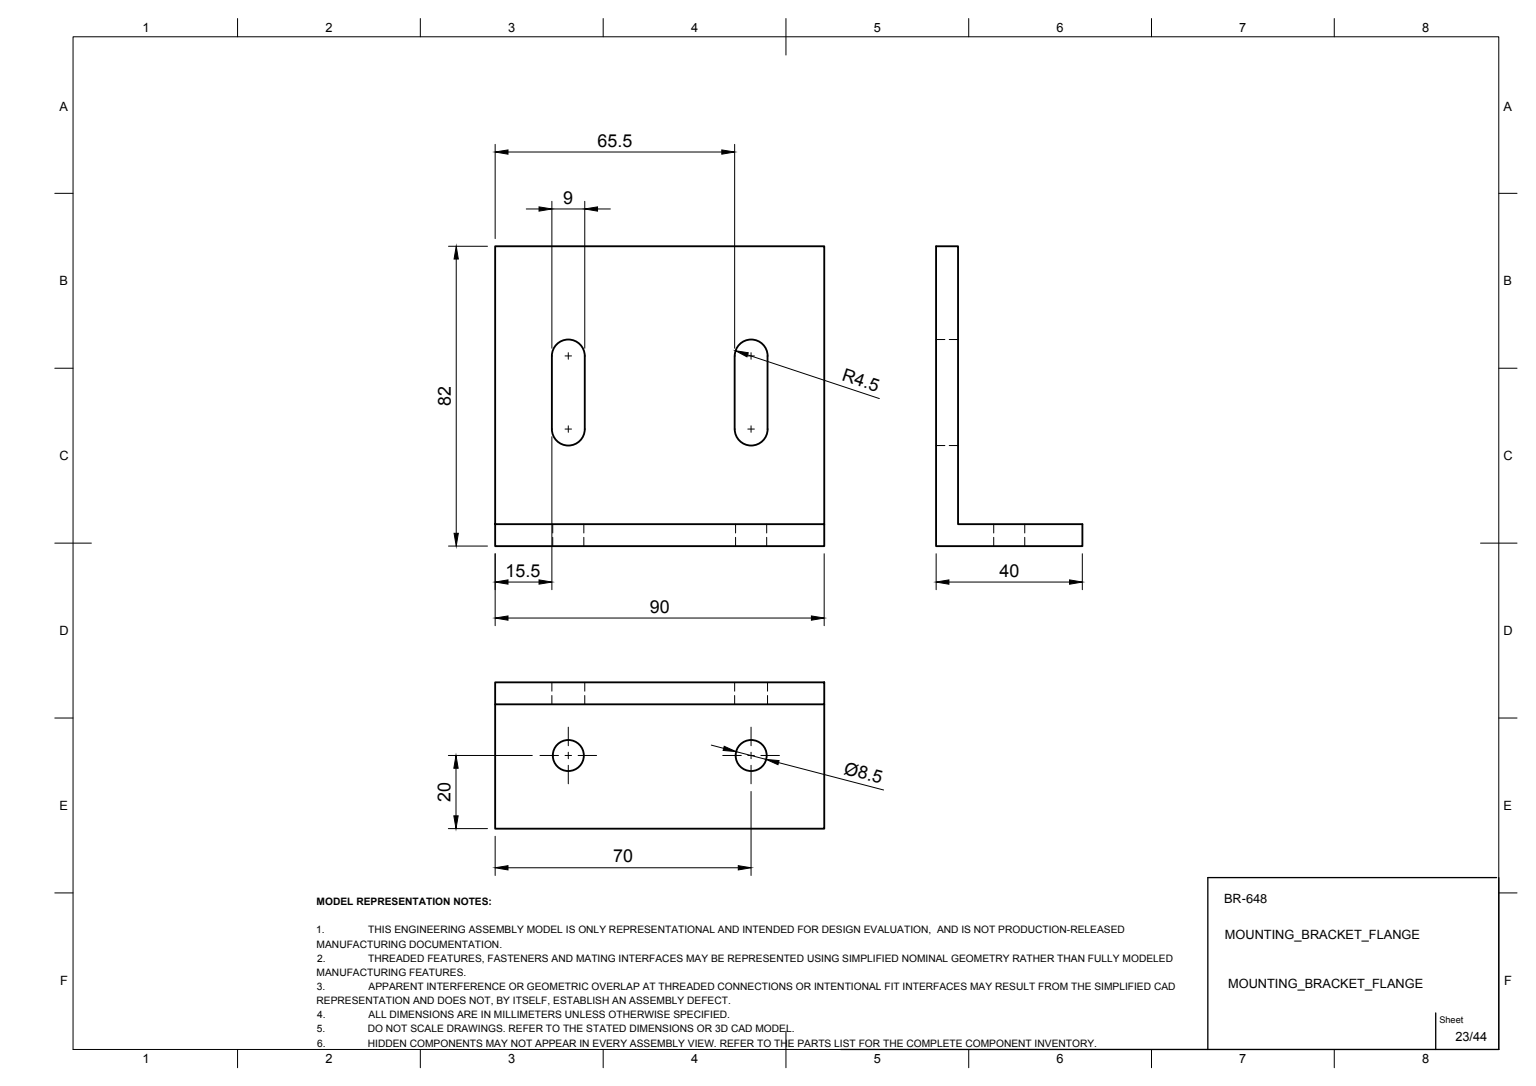
ISO-10303-21;
HEADER;
FILE_DESCRIPTION((''),'2;1');
FILE_NAME('MOUNTING_BRACKET_FLANGE.step','2026-10-01T22:05:39-07:00',(''),(''),'','','');
FILE_SCHEMA (('AUTOMOTIVE_DESIGN { 1 0 10303 214 3 1 1 }'));
ENDSEC;
DATA;
#10=MECHANICAL_DESIGN_GEOMETRIC_PRESENTATION_REPRESENTATION('',(#623),#24628);
#539=SHAPE_REPRESENTATION_RELATIONSHIP('SRR','None',#24811,#581) ;
#581=ADVANCED_BREP_SHAPE_REPRESENTATION('',(#662),#24601) ;
#623=STYLED_ITEM('',(#25037),#662) ;
#662=MANIFOLD_SOLID_BREP('MOUNTING_BRACKET_FLANGE',#13165) ;
#863=FACE_BOUND('',#4382,.T.) ;
#864=FACE_BOUND('',#4383,.T.) ;
#865=FACE_BOUND('',#4386,.T.) ;
#866=FACE_BOUND('',#4387,.T.) ;
#867=FACE_BOUND('',#4390,.T.) ;
#868=FACE_BOUND('',#4391,.T.) ;
#869=FACE_BOUND('',#4394,.T.) ;
#870=FACE_BOUND('',#4395,.T.) ;
#1406=LINE('',#22245,#2242) ;
#1407=LINE('',#22248,#2243) ;
#1408=LINE('',#22251,#2244) ;
#1409=LINE('',#22253,#2245) ;
#1410=LINE('',#22254,#2246) ;
#1411=LINE('',#22260,#2247) ;
#1412=LINE('',#22262,#2248) ;
#1413=LINE('',#22263,#2249) ;
#1414=LINE('',#22268,#2250) ;
#1415=LINE('',#22275,#2251) ;
#1416=LINE('',#22278,#2252) ;
#1417=LINE('',#22281,#2253) ;
#1418=LINE('',#22283,#2254) ;
#1419=LINE('',#22284,#2255) ;
#1420=LINE('',#22290,#2256) ;
#1421=LINE('',#22292,#2257) ;
#1422=LINE('',#22293,#2258) ;
#1423=LINE('',#22298,#2259) ;
#1424=LINE('',#22303,#2260) ;
#1425=LINE('',#22305,#2261) ;
#1426=LINE('',#22307,#2262) ;
#1427=LINE('',#22308,#2263) ;
#1428=LINE('',#22311,#2264) ;
#1429=LINE('',#22313,#2265) ;
#1430=LINE('',#22314,#2266) ;
#1431=LINE('',#22317,#2267) ;
#1432=LINE('',#22319,#2268) ;
#1433=LINE('',#22320,#2269) ;
#1434=LINE('',#22324,#2270) ;
#1435=LINE('',#22325,#2271) ;
#1436=LINE('',#22326,#2272) ;
#1437=LINE('',#22329,#2273) ;
#1438=LINE('',#22330,#2274) ;
#1439=LINE('',#22333,#2275) ;
#1440=LINE('',#22334,#2276) ;
#1441=LINE('',#22336,#2277) ;
#2242=VECTOR('',#18101,1.) ;
#2243=VECTOR('',#18104,1.) ;
#2244=VECTOR('',#18107,1.) ;
#2245=VECTOR('',#18108,1.) ;
#2246=VECTOR('',#18109,1.) ;
#2247=VECTOR('',#18116,1.) ;
#2248=VECTOR('',#18119,1.) ;
#2249=VECTOR('',#18120,1.) ;
#2250=VECTOR('',#18125,0.425) ;
#2251=VECTOR('',#18132,1.) ;
#2252=VECTOR('',#18135,1.) ;
#2253=VECTOR('',#18138,1.) ;
#2254=VECTOR('',#18139,1.) ;
#2255=VECTOR('',#18140,1.) ;
#2256=VECTOR('',#18147,1.) ;
#2257=VECTOR('',#18150,1.) ;
#2258=VECTOR('',#18151,1.) ;
#2259=VECTOR('',#18156,0.425) ;
#2260=VECTOR('',#18161,1.) ;
#2261=VECTOR('',#18162,1.) ;
#2262=VECTOR('',#18163,1.) ;
#2263=VECTOR('',#18164,1.) ;
#2264=VECTOR('',#18167,1.) ;
#2265=VECTOR('',#18168,1.) ;
#2266=VECTOR('',#18169,1.) ;
#2267=VECTOR('',#18172,1.) ;
#2268=VECTOR('',#18173,1.) ;
#2269=VECTOR('',#18174,1.) ;
#2270=VECTOR('',#18177,1.) ;
#2271=VECTOR('',#18178,1.) ;
#2272=VECTOR('',#18179,1.) ;
#2273=VECTOR('',#18182,1.) ;
#2274=VECTOR('',#18183,1.) ;
#2275=VECTOR('',#18186,1.) ;
#2276=VECTOR('',#18187,1.) ;
#2277=VECTOR('',#18190,1.) ;
#2868=CYLINDRICAL_SURFACE('',#14803,0.45) ;
#2869=CYLINDRICAL_SURFACE('',#14807,0.45) ;
#2870=CYLINDRICAL_SURFACE('',#14811,0.425) ;
#2871=CYLINDRICAL_SURFACE('',#14814,0.45) ;
#2872=CYLINDRICAL_SURFACE('',#14818,0.45) ;
#2873=CYLINDRICAL_SURFACE('',#14822,0.425) ;
#3427=FACE_OUTER_BOUND('',#4371,.T.) ;
#3428=FACE_OUTER_BOUND('',#4372,.T.) ;
#3429=FACE_OUTER_BOUND('',#4373,.T.) ;
#3430=FACE_OUTER_BOUND('',#4374,.T.) ;
#3431=FACE_OUTER_BOUND('',#4375,.T.) ;
#3432=FACE_OUTER_BOUND('',#4376,.T.) ;
#3433=FACE_OUTER_BOUND('',#4377,.T.) ;
#3434=FACE_OUTER_BOUND('',#4378,.T.) ;
#3435=FACE_OUTER_BOUND('',#4379,.T.) ;
#3436=FACE_OUTER_BOUND('',#4380,.T.) ;
#3437=FACE_OUTER_BOUND('',#4381,.T.) ;
#3438=FACE_OUTER_BOUND('',#4384,.T.) ;
#3439=FACE_OUTER_BOUND('',#4385,.T.) ;
#3440=FACE_OUTER_BOUND('',#4388,.T.) ;
#3441=FACE_OUTER_BOUND('',#4389,.T.) ;
#3442=FACE_OUTER_BOUND('',#4392,.T.) ;
#3443=FACE_OUTER_BOUND('',#4393,.T.) ;
#3444=FACE_OUTER_BOUND('',#4396,.T.) ;
#4371=EDGE_LOOP('',(#10633,#10634,#10635,#10636)) ;
#4372=EDGE_LOOP('',(#10637,#10638,#10639,#10640)) ;
#4373=EDGE_LOOP('',(#10641,#10642,#10643,#10644)) ;
#4374=EDGE_LOOP('',(#10645,#10646,#10647,#10648)) ;
#4375=EDGE_LOOP('',(#10649,#10650,#10651,#10652)) ;
#4376=EDGE_LOOP('',(#10653,#10654,#10655,#10656)) ;
#4377=EDGE_LOOP('',(#10657,#10658,#10659,#10660)) ;
#4378=EDGE_LOOP('',(#10661,#10662,#10663,#10664)) ;
#4379=EDGE_LOOP('',(#10665,#10666,#10667,#10668)) ;
#4380=EDGE_LOOP('',(#10669,#10670,#10671,#10672)) ;
#4381=EDGE_LOOP('',(#10673,#10674,#10675,#10676)) ;
#4382=EDGE_LOOP('',(#10677,#10678,#10679,#10680)) ;
#4383=EDGE_LOOP('',(#10681,#10682,#10683,#10684)) ;
#4384=EDGE_LOOP('',(#10685,#10686,#10687,#10688)) ;
#4385=EDGE_LOOP('',(#10689,#10690,#10691,#10692)) ;
#4386=EDGE_LOOP('',(#10693)) ;
#4387=EDGE_LOOP('',(#10694)) ;
#4388=EDGE_LOOP('',(#10695,#10696,#10697,#10698,#10699,#10700)) ;
#4389=EDGE_LOOP('',(#10701,#10702,#10703,#10704)) ;
#4390=EDGE_LOOP('',(#10705,#10706,#10707,#10708)) ;
#4391=EDGE_LOOP('',(#10709,#10710,#10711,#10712)) ;
#4392=EDGE_LOOP('',(#10713,#10714,#10715,#10716)) ;
#4393=EDGE_LOOP('',(#10717,#10718,#10719,#10720)) ;
#4394=EDGE_LOOP('',(#10721)) ;
#4395=EDGE_LOOP('',(#10722)) ;
#4396=EDGE_LOOP('',(#10723,#10724,#10725,#10726,#10727,#10728)) ;
#5330=CIRCLE('',#14804,0.45) ;
#5331=CIRCLE('',#14805,0.45) ;
#5332=CIRCLE('',#14808,0.45) ;
#5333=CIRCLE('',#14809,0.45) ;
#5334=CIRCLE('',#14812,0.425) ;
#5335=CIRCLE('',#14813,0.425) ;
#5336=CIRCLE('',#14815,0.45) ;
#5337=CIRCLE('',#14816,0.45) ;
#5338=CIRCLE('',#14819,0.45) ;
#5339=CIRCLE('',#14820,0.45) ;
#5340=CIRCLE('',#14823,0.425) ;
#5341=CIRCLE('',#14824,0.425) ;
#6280=VERTEX_POINT('',#22241) ;
#6281=VERTEX_POINT('',#22242) ;
#6282=VERTEX_POINT('',#22244) ;
#6283=VERTEX_POINT('',#22246) ;
#6284=VERTEX_POINT('',#22250) ;
#6285=VERTEX_POINT('',#22252) ;
#6286=VERTEX_POINT('',#22256) ;
#6287=VERTEX_POINT('',#22258) ;
#6288=VERTEX_POINT('',#22265) ;
#6289=VERTEX_POINT('',#22267) ;
#6290=VERTEX_POINT('',#22271) ;
#6291=VERTEX_POINT('',#22272) ;
#6292=VERTEX_POINT('',#22274) ;
#6293=VERTEX_POINT('',#22276) ;
#6294=VERTEX_POINT('',#22280) ;
#6295=VERTEX_POINT('',#22282) ;
#6296=VERTEX_POINT('',#22286) ;
#6297=VERTEX_POINT('',#22288) ;
#6298=VERTEX_POINT('',#22295) ;
#6299=VERTEX_POINT('',#22297) ;
#6300=VERTEX_POINT('',#22301) ;
#6301=VERTEX_POINT('',#22302) ;
#6302=VERTEX_POINT('',#22304) ;
#6303=VERTEX_POINT('',#22306) ;
#6304=VERTEX_POINT('',#22310) ;
#6305=VERTEX_POINT('',#22312) ;
#6306=VERTEX_POINT('',#22316) ;
#6307=VERTEX_POINT('',#22318) ;
#6308=VERTEX_POINT('',#22322) ;
#6309=VERTEX_POINT('',#22323) ;
#6310=VERTEX_POINT('',#22328) ;
#6311=VERTEX_POINT('',#22332) ;
#7806=EDGE_CURVE('',#6280,#6281,#5330,.T.) ;
#7807=EDGE_CURVE('',#6282,#6280,#1406,.T.) ;
#7808=EDGE_CURVE('',#6283,#6282,#5331,.T.) ;
#7809=EDGE_CURVE('',#6283,#6281,#1407,.T.) ;
#7810=EDGE_CURVE('',#6281,#6284,#1408,.T.) ;
#7811=EDGE_CURVE('',#6285,#6283,#1409,.T.) ;
#7812=EDGE_CURVE('',#6285,#6284,#1410,.T.) ;
#7813=EDGE_CURVE('',#6284,#6286,#5332,.T.) ;
#7814=EDGE_CURVE('',#6287,#6285,#5333,.T.) ;
#7815=EDGE_CURVE('',#6287,#6286,#1411,.T.) ;
#7816=EDGE_CURVE('',#6286,#6280,#1412,.T.) ;
#7817=EDGE_CURVE('',#6282,#6287,#1413,.T.) ;
#7818=EDGE_CURVE('',#6288,#6288,#5334,.T.) ;
#7819=EDGE_CURVE('',#6288,#6289,#1414,.T.) ;
#7820=EDGE_CURVE('',#6289,#6289,#5335,.T.) ;
#7821=EDGE_CURVE('',#6290,#6291,#5336,.T.) ;
#7822=EDGE_CURVE('',#6292,#6290,#1415,.T.) ;
#7823=EDGE_CURVE('',#6293,#6292,#5337,.T.) ;
#7824=EDGE_CURVE('',#6293,#6291,#1416,.T.) ;
#7825=EDGE_CURVE('',#6291,#6294,#1417,.T.) ;
#7826=EDGE_CURVE('',#6295,#6293,#1418,.T.) ;
#7827=EDGE_CURVE('',#6295,#6294,#1419,.T.) ;
#7828=EDGE_CURVE('',#6294,#6296,#5338,.T.) ;
#7829=EDGE_CURVE('',#6297,#6295,#5339,.T.) ;
#7830=EDGE_CURVE('',#6297,#6296,#1420,.T.) ;
#7831=EDGE_CURVE('',#6296,#6290,#1421,.T.) ;
#7832=EDGE_CURVE('',#6292,#6297,#1422,.T.) ;
#7833=EDGE_CURVE('',#6298,#6298,#5340,.T.) ;
#7834=EDGE_CURVE('',#6298,#6299,#1423,.T.) ;
#7835=EDGE_CURVE('',#6299,#6299,#5341,.T.) ;
#7836=EDGE_CURVE('',#6300,#6301,#1424,.T.) ;
#7837=EDGE_CURVE('',#6300,#6302,#1425,.T.) ;
#7838=EDGE_CURVE('',#6302,#6303,#1426,.T.) ;
#7839=EDGE_CURVE('',#6303,#6301,#1427,.T.) ;
#7840=EDGE_CURVE('',#6304,#6303,#1428,.T.) ;
#7841=EDGE_CURVE('',#6305,#6302,#1429,.T.) ;
#7842=EDGE_CURVE('',#6304,#6305,#1430,.T.) ;
#7843=EDGE_CURVE('',#6301,#6306,#1431,.T.) ;
#7844=EDGE_CURVE('',#6307,#6306,#1432,.T.) ;
#7845=EDGE_CURVE('',#6300,#6307,#1433,.T.) ;
#7846=EDGE_CURVE('',#6308,#6309,#1434,.T.) ;
#7847=EDGE_CURVE('',#6306,#6309,#1435,.T.) ;
#7848=EDGE_CURVE('',#6308,#6304,#1436,.T.) ;
#7849=EDGE_CURVE('',#6305,#6310,#1437,.T.) ;
#7850=EDGE_CURVE('',#6310,#6308,#1438,.T.) ;
#7851=EDGE_CURVE('',#6309,#6311,#1439,.T.) ;
#7852=EDGE_CURVE('',#6311,#6307,#1440,.T.) ;
#7853=EDGE_CURVE('',#6310,#6311,#1441,.T.) ;
#10633=ORIENTED_EDGE('',*,*,#7806,.F.) ;
#10634=ORIENTED_EDGE('',*,*,#7807,.F.) ;
#10635=ORIENTED_EDGE('',*,*,#7808,.F.) ;
#10636=ORIENTED_EDGE('',*,*,#7809,.T.) ;
#10637=ORIENTED_EDGE('',*,*,#7810,.F.) ;
#10638=ORIENTED_EDGE('',*,*,#7809,.F.) ;
#10639=ORIENTED_EDGE('',*,*,#7811,.F.) ;
#10640=ORIENTED_EDGE('',*,*,#7812,.T.) ;
#10641=ORIENTED_EDGE('',*,*,#7813,.F.) ;
#10642=ORIENTED_EDGE('',*,*,#7812,.F.) ;
#10643=ORIENTED_EDGE('',*,*,#7814,.F.) ;
#10644=ORIENTED_EDGE('',*,*,#7815,.T.) ;
#10645=ORIENTED_EDGE('',*,*,#7816,.F.) ;
#10646=ORIENTED_EDGE('',*,*,#7815,.F.) ;
#10647=ORIENTED_EDGE('',*,*,#7817,.F.) ;
#10648=ORIENTED_EDGE('',*,*,#7807,.T.) ;
#10649=ORIENTED_EDGE('',*,*,#7818,.F.) ;
#10650=ORIENTED_EDGE('',*,*,#7819,.T.) ;
#10651=ORIENTED_EDGE('',*,*,#7820,.F.) ;
#10652=ORIENTED_EDGE('',*,*,#7819,.F.) ;
#10653=ORIENTED_EDGE('',*,*,#7821,.F.) ;
#10654=ORIENTED_EDGE('',*,*,#7822,.F.) ;
#10655=ORIENTED_EDGE('',*,*,#7823,.F.) ;
#10656=ORIENTED_EDGE('',*,*,#7824,.T.) ;
#10657=ORIENTED_EDGE('',*,*,#7825,.F.) ;
#10658=ORIENTED_EDGE('',*,*,#7824,.F.) ;
#10659=ORIENTED_EDGE('',*,*,#7826,.F.) ;
#10660=ORIENTED_EDGE('',*,*,#7827,.T.) ;
#10661=ORIENTED_EDGE('',*,*,#7828,.F.) ;
#10662=ORIENTED_EDGE('',*,*,#7827,.F.) ;
#10663=ORIENTED_EDGE('',*,*,#7829,.F.) ;
#10664=ORIENTED_EDGE('',*,*,#7830,.T.) ;
#10665=ORIENTED_EDGE('',*,*,#7831,.F.) ;
#10666=ORIENTED_EDGE('',*,*,#7830,.F.) ;
#10667=ORIENTED_EDGE('',*,*,#7832,.F.) ;
#10668=ORIENTED_EDGE('',*,*,#7822,.T.) ;
#10669=ORIENTED_EDGE('',*,*,#7833,.F.) ;
#10670=ORIENTED_EDGE('',*,*,#7834,.T.) ;
#10671=ORIENTED_EDGE('',*,*,#7835,.F.) ;
#10672=ORIENTED_EDGE('',*,*,#7834,.F.) ;
#10673=ORIENTED_EDGE('',*,*,#7836,.F.) ;
#10674=ORIENTED_EDGE('',*,*,#7837,.T.) ;
#10675=ORIENTED_EDGE('',*,*,#7838,.T.) ;
#10676=ORIENTED_EDGE('',*,*,#7839,.T.) ;
#10677=ORIENTED_EDGE('',*,*,#7813,.T.) ;
#10678=ORIENTED_EDGE('',*,*,#7816,.T.) ;
#10679=ORIENTED_EDGE('',*,*,#7806,.T.) ;
#10680=ORIENTED_EDGE('',*,*,#7810,.T.) ;
#10681=ORIENTED_EDGE('',*,*,#7828,.T.) ;
#10682=ORIENTED_EDGE('',*,*,#7831,.T.) ;
#10683=ORIENTED_EDGE('',*,*,#7821,.T.) ;
#10684=ORIENTED_EDGE('',*,*,#7825,.T.) ;
#10685=ORIENTED_EDGE('',*,*,#7840,.T.) ;
#10686=ORIENTED_EDGE('',*,*,#7838,.F.) ;
#10687=ORIENTED_EDGE('',*,*,#7841,.F.) ;
#10688=ORIENTED_EDGE('',*,*,#7842,.F.) ;
#10689=ORIENTED_EDGE('',*,*,#7836,.T.) ;
#10690=ORIENTED_EDGE('',*,*,#7843,.T.) ;
#10691=ORIENTED_EDGE('',*,*,#7844,.F.) ;
#10692=ORIENTED_EDGE('',*,*,#7845,.F.) ;
#10693=ORIENTED_EDGE('',*,*,#7820,.T.) ;
#10694=ORIENTED_EDGE('',*,*,#7835,.T.) ;
#10695=ORIENTED_EDGE('',*,*,#7846,.T.) ;
#10696=ORIENTED_EDGE('',*,*,#7847,.F.) ;
#10697=ORIENTED_EDGE('',*,*,#7843,.F.) ;
#10698=ORIENTED_EDGE('',*,*,#7839,.F.) ;
#10699=ORIENTED_EDGE('',*,*,#7840,.F.) ;
#10700=ORIENTED_EDGE('',*,*,#7848,.F.) ;
#10701=ORIENTED_EDGE('',*,*,#7848,.T.) ;
#10702=ORIENTED_EDGE('',*,*,#7842,.T.) ;
#10703=ORIENTED_EDGE('',*,*,#7849,.T.) ;
#10704=ORIENTED_EDGE('',*,*,#7850,.T.) ;
#10705=ORIENTED_EDGE('',*,*,#7814,.T.) ;
#10706=ORIENTED_EDGE('',*,*,#7811,.T.) ;
#10707=ORIENTED_EDGE('',*,*,#7808,.T.) ;
#10708=ORIENTED_EDGE('',*,*,#7817,.T.) ;
#10709=ORIENTED_EDGE('',*,*,#7829,.T.) ;
#10710=ORIENTED_EDGE('',*,*,#7826,.T.) ;
#10711=ORIENTED_EDGE('',*,*,#7823,.T.) ;
#10712=ORIENTED_EDGE('',*,*,#7832,.T.) ;
#10713=ORIENTED_EDGE('',*,*,#7847,.T.) ;
#10714=ORIENTED_EDGE('',*,*,#7851,.T.) ;
#10715=ORIENTED_EDGE('',*,*,#7852,.T.) ;
#10716=ORIENTED_EDGE('',*,*,#7844,.T.) ;
#10717=ORIENTED_EDGE('',*,*,#7853,.T.) ;
#10718=ORIENTED_EDGE('',*,*,#7851,.F.) ;
#10719=ORIENTED_EDGE('',*,*,#7846,.F.) ;
#10720=ORIENTED_EDGE('',*,*,#7850,.F.) ;
#10721=ORIENTED_EDGE('',*,*,#7818,.T.) ;
#10722=ORIENTED_EDGE('',*,*,#7833,.T.) ;
#10723=ORIENTED_EDGE('',*,*,#7845,.T.) ;
#10724=ORIENTED_EDGE('',*,*,#7852,.F.) ;
#10725=ORIENTED_EDGE('',*,*,#7853,.F.) ;
#10726=ORIENTED_EDGE('',*,*,#7849,.F.) ;
#10727=ORIENTED_EDGE('',*,*,#7841,.T.) ;
#10728=ORIENTED_EDGE('',*,*,#7837,.F.) ;
#12152=PLANE('',#14806) ;
#12153=PLANE('',#14810) ;
#12154=PLANE('',#14817) ;
#12155=PLANE('',#14821) ;
#12156=PLANE('',#14825) ;
#12157=PLANE('',#14826) ;
#12158=PLANE('',#14827) ;
#12159=PLANE('',#14828) ;
#12160=PLANE('',#14829) ;
#12161=PLANE('',#14830) ;
#12162=PLANE('',#14831) ;
#12163=PLANE('',#14832) ;
#12822=ADVANCED_FACE('',(#3427),#2868,.F.) ;
#12823=ADVANCED_FACE('',(#3428),#12152,.T.) ;
#12824=ADVANCED_FACE('',(#3429),#2869,.F.) ;
#12825=ADVANCED_FACE('',(#3430),#12153,.T.) ;
#12826=ADVANCED_FACE('',(#3431),#2870,.F.) ;
#12827=ADVANCED_FACE('',(#3432),#2871,.F.) ;
#12828=ADVANCED_FACE('',(#3433),#12154,.T.) ;
#12829=ADVANCED_FACE('',(#3434),#2872,.F.) ;
#12830=ADVANCED_FACE('',(#3435),#12155,.T.) ;
#12831=ADVANCED_FACE('',(#3436),#2873,.F.) ;
#12832=ADVANCED_FACE('',(#3437,#863,#864),#12156,.F.) ;
#12833=ADVANCED_FACE('',(#3438),#12157,.F.) ;
#12834=ADVANCED_FACE('',(#3439,#865,#866),#12158,.F.) ;
#12835=ADVANCED_FACE('',(#3440),#12159,.F.) ;
#12836=ADVANCED_FACE('',(#3441,#867,#868),#12160,.T.) ;
#12837=ADVANCED_FACE('',(#3442),#12161,.F.) ;
#12838=ADVANCED_FACE('',(#3443,#869,#870),#12162,.F.) ;
#12839=ADVANCED_FACE('',(#3444),#12163,.F.) ;
#13165=CLOSED_SHELL('',(#12822,#12823,#12824,#12825,#12826,#12827,#12828,
#12829,#12830,#12831,#12832,#12833,#12834,#12835,#12836,#12837,#12838,#12839)) ;
#14802=AXIS2_PLACEMENT_3D('',#22239,#18095,#18096) ;
#14803=AXIS2_PLACEMENT_3D('',#22240,#18097,#18098) ;
#14804=AXIS2_PLACEMENT_3D('',#22243,#18099,#18100) ;
#14805=AXIS2_PLACEMENT_3D('',#22247,#18102,#18103) ;
#14806=AXIS2_PLACEMENT_3D('',#22249,#18105,#18106) ;
#14807=AXIS2_PLACEMENT_3D('',#22255,#18110,#18111) ;
#14808=AXIS2_PLACEMENT_3D('',#22257,#18112,#18113) ;
#14809=AXIS2_PLACEMENT_3D('',#22259,#18114,#18115) ;
#14810=AXIS2_PLACEMENT_3D('',#22261,#18117,#18118) ;
#14811=AXIS2_PLACEMENT_3D('',#22264,#18121,#18122) ;
#14812=AXIS2_PLACEMENT_3D('',#22266,#18123,#18124) ;
#14813=AXIS2_PLACEMENT_3D('',#22269,#18126,#18127) ;
#14814=AXIS2_PLACEMENT_3D('',#22270,#18128,#18129) ;
#14815=AXIS2_PLACEMENT_3D('',#22273,#18130,#18131) ;
#14816=AXIS2_PLACEMENT_3D('',#22277,#18133,#18134) ;
#14817=AXIS2_PLACEMENT_3D('',#22279,#18136,#18137) ;
#14818=AXIS2_PLACEMENT_3D('',#22285,#18141,#18142) ;
#14819=AXIS2_PLACEMENT_3D('',#22287,#18143,#18144) ;
#14820=AXIS2_PLACEMENT_3D('',#22289,#18145,#18146) ;
#14821=AXIS2_PLACEMENT_3D('',#22291,#18148,#18149) ;
#14822=AXIS2_PLACEMENT_3D('',#22294,#18152,#18153) ;
#14823=AXIS2_PLACEMENT_3D('',#22296,#18154,#18155) ;
#14824=AXIS2_PLACEMENT_3D('',#22299,#18157,#18158) ;
#14825=AXIS2_PLACEMENT_3D('',#22300,#18159,#18160) ;
#14826=AXIS2_PLACEMENT_3D('',#22309,#18165,#18166) ;
#14827=AXIS2_PLACEMENT_3D('',#22315,#18170,#18171) ;
#14828=AXIS2_PLACEMENT_3D('',#22321,#18175,#18176) ;
#14829=AXIS2_PLACEMENT_3D('',#22327,#18180,#18181) ;
#14830=AXIS2_PLACEMENT_3D('',#22331,#18184,#18185) ;
#14831=AXIS2_PLACEMENT_3D('',#22335,#18188,#18189) ;
#14832=AXIS2_PLACEMENT_3D('',#22337,#18191,#18192) ;
#18095=DIRECTION('axis',(0.,0.,1.)) ;
#18096=DIRECTION('refdir',(1.,0.,0.)) ;
#18097=DIRECTION('center_axis',(0.,0.,1.)) ;
#18098=DIRECTION('ref_axis',(1.,0.,0.)) ;
#18099=DIRECTION('center_axis',(0.,0.,1.)) ;
#18100=DIRECTION('ref_axis',(1.,0.,0.)) ;
#18101=DIRECTION('',(0.,0.,-1.)) ;
#18102=DIRECTION('center_axis',(0.,0.,-1.)) ;
#18103=DIRECTION('ref_axis',(1.,0.,0.)) ;
#18104=DIRECTION('',(0.,0.,-1.)) ;
#18105=DIRECTION('center_axis',(-1.,0.,0.)) ;
#18106=DIRECTION('ref_axis',(0.,0.,1.)) ;
#18107=DIRECTION('',(0.,1.,0.)) ;
#18108=DIRECTION('',(0.,-1.,0.)) ;
#18109=DIRECTION('',(0.,0.,-1.)) ;
#18110=DIRECTION('center_axis',(0.,0.,1.)) ;
#18111=DIRECTION('ref_axis',(1.,0.,0.)) ;
#18112=DIRECTION('center_axis',(0.,0.,1.)) ;
#18113=DIRECTION('ref_axis',(1.,0.,0.)) ;
#18114=DIRECTION('center_axis',(0.,0.,-1.)) ;
#18115=DIRECTION('ref_axis',(1.,0.,0.)) ;
#18116=DIRECTION('',(0.,0.,-1.)) ;
#18117=DIRECTION('center_axis',(1.,0.,0.)) ;
#18118=DIRECTION('ref_axis',(0.,0.,-1.)) ;
#18119=DIRECTION('',(0.,-1.,0.)) ;
#18120=DIRECTION('',(0.,1.,0.)) ;
#18121=DIRECTION('center_axis',(0.,1.,0.)) ;
#18122=DIRECTION('ref_axis',(1.,0.,0.)) ;
#18123=DIRECTION('center_axis',(0.,1.,0.)) ;
#18124=DIRECTION('ref_axis',(1.,0.,0.)) ;
#18125=DIRECTION('',(0.,1.,0.)) ;
#18126=DIRECTION('center_axis',(0.,-1.,0.)) ;
#18127=DIRECTION('ref_axis',(1.,0.,0.)) ;
#18128=DIRECTION('center_axis',(0.,0.,1.)) ;
#18129=DIRECTION('ref_axis',(1.,0.,0.)) ;
#18130=DIRECTION('center_axis',(0.,0.,1.)) ;
#18131=DIRECTION('ref_axis',(1.,0.,0.)) ;
#18132=DIRECTION('',(0.,0.,-1.)) ;
#18133=DIRECTION('center_axis',(0.,0.,-1.)) ;
#18134=DIRECTION('ref_axis',(1.,0.,0.)) ;
#18135=DIRECTION('',(0.,0.,-1.)) ;
#18136=DIRECTION('center_axis',(-1.,0.,0.)) ;
#18137=DIRECTION('ref_axis',(0.,0.,1.)) ;
#18138=DIRECTION('',(0.,1.,0.)) ;
#18139=DIRECTION('',(0.,-1.,0.)) ;
#18140=DIRECTION('',(0.,0.,-1.)) ;
#18141=DIRECTION('center_axis',(0.,0.,1.)) ;
#18142=DIRECTION('ref_axis',(1.,0.,0.)) ;
#18143=DIRECTION('center_axis',(0.,0.,1.)) ;
#18144=DIRECTION('ref_axis',(1.,0.,0.)) ;
#18145=DIRECTION('center_axis',(0.,0.,-1.)) ;
#18146=DIRECTION('ref_axis',(1.,0.,0.)) ;
#18147=DIRECTION('',(0.,0.,-1.)) ;
#18148=DIRECTION('center_axis',(1.,0.,0.)) ;
#18149=DIRECTION('ref_axis',(0.,0.,-1.)) ;
#18150=DIRECTION('',(0.,-1.,0.)) ;
#18151=DIRECTION('',(0.,1.,0.)) ;
#18152=DIRECTION('center_axis',(0.,1.,0.)) ;
#18153=DIRECTION('ref_axis',(1.,0.,0.)) ;
#18154=DIRECTION('center_axis',(0.,1.,0.)) ;
#18155=DIRECTION('ref_axis',(1.,0.,0.)) ;
#18156=DIRECTION('',(0.,1.,0.)) ;
#18157=DIRECTION('center_axis',(0.,-1.,0.)) ;
#18158=DIRECTION('ref_axis',(1.,0.,0.)) ;
#18159=DIRECTION('center_axis',(0.,0.,1.)) ;
#18160=DIRECTION('ref_axis',(1.,0.,0.)) ;
#18161=DIRECTION('',(1.,0.,0.)) ;
#18162=DIRECTION('',(0.,1.,0.)) ;
#18163=DIRECTION('',(1.,0.,0.)) ;
#18164=DIRECTION('',(0.,-1.,0.)) ;
#18165=DIRECTION('center_axis',(0.,-1.,0.)) ;
#18166=DIRECTION('ref_axis',(0.,0.,-1.)) ;
#18167=DIRECTION('',(0.,0.,-1.)) ;
#18168=DIRECTION('',(0.,0.,-1.)) ;
#18169=DIRECTION('',(-1.,0.,0.)) ;
#18170=DIRECTION('center_axis',(0.,-1.,0.)) ;
#18171=DIRECTION('ref_axis',(0.,0.,-1.)) ;
#18172=DIRECTION('',(0.,0.,-1.)) ;
#18173=DIRECTION('',(1.,0.,0.)) ;
#18174=DIRECTION('',(0.,0.,-1.)) ;
#18175=DIRECTION('center_axis',(-1.,0.,0.)) ;
#18176=DIRECTION('ref_axis',(0.,0.,1.)) ;
#18177=DIRECTION('',(0.,0.,-1.)) ;
#18178=DIRECTION('',(0.,-1.,0.)) ;
#18179=DIRECTION('',(0.,1.,0.)) ;
#18180=DIRECTION('center_axis',(0.,0.,1.)) ;
#18181=DIRECTION('ref_axis',(1.,0.,0.)) ;
#18182=DIRECTION('',(0.,-1.,0.)) ;
#18183=DIRECTION('',(1.,0.,0.)) ;
#18184=DIRECTION('center_axis',(0.,0.,1.)) ;
#18185=DIRECTION('ref_axis',(1.,0.,0.)) ;
#18186=DIRECTION('',(-1.,0.,0.)) ;
#18187=DIRECTION('',(0.,1.,0.)) ;
#18188=DIRECTION('center_axis',(0.,1.,0.)) ;
#18189=DIRECTION('ref_axis',(0.,0.,1.)) ;
#18190=DIRECTION('',(0.,0.,-1.)) ;
#18191=DIRECTION('center_axis',(1.,0.,0.)) ;
#18192=DIRECTION('ref_axis',(0.,0.,-1.)) ;
#22239=CARTESIAN_POINT('',(0.,0.,0.)) ;
#22240=CARTESIAN_POINT('Origin',(2.5,-2.,13.2)) ;
#22241=CARTESIAN_POINT('',(2.05,-2.,12.9)) ;
#22242=CARTESIAN_POINT('',(2.95,-2.,12.9)) ;
#22243=CARTESIAN_POINT('Origin',(2.5,-2.,12.9)) ;
#22244=CARTESIAN_POINT('',(2.05,-2.,13.5)) ;
#22245=CARTESIAN_POINT('',(2.05,-2.,13.2)) ;
#22246=CARTESIAN_POINT('',(2.95,-2.,13.5)) ;
#22247=CARTESIAN_POINT('Origin',(2.5,-2.,13.5)) ;
#22248=CARTESIAN_POINT('',(2.95,-2.,13.2)) ;
#22249=CARTESIAN_POINT('Origin',(2.95,-1.,13.2)) ;
#22250=CARTESIAN_POINT('',(2.95,0.,12.9)) ;
#22251=CARTESIAN_POINT('',(2.95,-1.05,12.9)) ;
#22252=CARTESIAN_POINT('',(2.95,0.,13.5)) ;
#22253=CARTESIAN_POINT('',(2.95,-2.95,13.5)) ;
#22254=CARTESIAN_POINT('',(2.95,0.,13.2)) ;
#22255=CARTESIAN_POINT('Origin',(2.5,0.,13.2)) ;
#22256=CARTESIAN_POINT('',(2.05,0.,12.9)) ;
#22257=CARTESIAN_POINT('Origin',(2.5,0.,12.9)) ;
#22258=CARTESIAN_POINT('',(2.05,0.,13.5)) ;
#22259=CARTESIAN_POINT('Origin',(2.5,0.,13.5)) ;
#22260=CARTESIAN_POINT('',(2.05,0.,13.2)) ;
#22261=CARTESIAN_POINT('Origin',(2.05,-1.,13.2)) ;
#22262=CARTESIAN_POINT('',(2.05,-1.05,12.9)) ;
#22263=CARTESIAN_POINT('',(2.05,-2.95,13.5)) ;
#22264=CARTESIAN_POINT('Origin',(2.5,-4.9,11.5)) ;
#22265=CARTESIAN_POINT('',(2.075,-5.2,11.5)) ;
#22266=CARTESIAN_POINT('Origin',(2.5,-5.2,11.5)) ;
#22267=CARTESIAN_POINT('',(2.075,-4.6,11.5)) ;
#22268=CARTESIAN_POINT('',(2.075,-4.9,11.5)) ;
#22269=CARTESIAN_POINT('Origin',(2.5,-4.6,11.5)) ;
#22270=CARTESIAN_POINT('Origin',(-2.5,-2.,13.2)) ;
#22271=CARTESIAN_POINT('',(-2.95,-2.,12.9)) ;
#22272=CARTESIAN_POINT('',(-2.05,-2.,12.9)) ;
#22273=CARTESIAN_POINT('Origin',(-2.5,-2.,12.9)) ;
#22274=CARTESIAN_POINT('',(-2.95,-2.,13.5)) ;
#22275=CARTESIAN_POINT('',(-2.95,-2.,13.2)) ;
#22276=CARTESIAN_POINT('',(-2.05,-2.,13.5)) ;
#22277=CARTESIAN_POINT('Origin',(-2.5,-2.,13.5)) ;
#22278=CARTESIAN_POINT('',(-2.05,-2.,13.2)) ;
#22279=CARTESIAN_POINT('Origin',(-2.05,-1.,13.2)) ;
#22280=CARTESIAN_POINT('',(-2.05,0.,12.9)) ;
#22281=CARTESIAN_POINT('',(-2.05,-1.05,12.9)) ;
#22282=CARTESIAN_POINT('',(-2.05,0.,13.5)) ;
#22283=CARTESIAN_POINT('',(-2.05,-2.95,13.5)) ;
#22284=CARTESIAN_POINT('',(-2.05,0.,13.2)) ;
#22285=CARTESIAN_POINT('Origin',(-2.5,0.,13.2)) ;
#22286=CARTESIAN_POINT('',(-2.95,0.,12.9)) ;
#22287=CARTESIAN_POINT('Origin',(-2.5,0.,12.9)) ;
#22288=CARTESIAN_POINT('',(-2.95,0.,13.5)) ;
#22289=CARTESIAN_POINT('Origin',(-2.5,0.,13.5)) ;
#22290=CARTESIAN_POINT('',(-2.95,0.,13.2)) ;
#22291=CARTESIAN_POINT('Origin',(-2.95,-1.,13.2)) ;
#22292=CARTESIAN_POINT('',(-2.95,-1.05,12.9)) ;
#22293=CARTESIAN_POINT('',(-2.95,-2.95,13.5)) ;
#22294=CARTESIAN_POINT('Origin',(-2.5,-4.9,11.5)) ;
#22295=CARTESIAN_POINT('',(-2.925,-5.2,11.5)) ;
#22296=CARTESIAN_POINT('Origin',(-2.5,-5.2,11.5)) ;
#22297=CARTESIAN_POINT('',(-2.925,-4.6,11.5)) ;
#22298=CARTESIAN_POINT('',(-2.925,-4.9,11.5)) ;
#22299=CARTESIAN_POINT('Origin',(-2.5,-4.6,11.5)) ;
#22300=CARTESIAN_POINT('Origin',(0.,-1.1,12.9)) ;
#22301=CARTESIAN_POINT('',(-4.5,-4.6,12.9)) ;
#22302=CARTESIAN_POINT('',(4.5,-4.6,12.9)) ;
#22303=CARTESIAN_POINT('',(0.,-4.6,12.9)) ;
#22304=CARTESIAN_POINT('',(-4.5,3.,12.9)) ;
#22305=CARTESIAN_POINT('',(-4.5,-1.1,12.9)) ;
#22306=CARTESIAN_POINT('',(4.5,3.,12.9)) ;
#22307=CARTESIAN_POINT('',(0.,3.,12.9)) ;
#22308=CARTESIAN_POINT('',(4.5,-1.1,12.9)) ;
#22309=CARTESIAN_POINT('Origin',(0.,3.,13.2)) ;
#22310=CARTESIAN_POINT('',(4.5,3.,13.5)) ;
#22311=CARTESIAN_POINT('',(4.5,3.,13.2)) ;
#22312=CARTESIAN_POINT('',(-4.5,3.,13.5)) ;
#22313=CARTESIAN_POINT('',(-4.5,3.,13.2)) ;
#22314=CARTESIAN_POINT('',(0.,3.,13.5)) ;
#22315=CARTESIAN_POINT('Origin',(0.,-4.6,11.5)) ;
#22316=CARTESIAN_POINT('',(4.5,-4.6,9.5)) ;
#22317=CARTESIAN_POINT('',(4.5,-4.6,11.5)) ;
#22318=CARTESIAN_POINT('',(-4.5,-4.6,9.5)) ;
#22319=CARTESIAN_POINT('',(0.,-4.6,9.5)) ;
#22320=CARTESIAN_POINT('',(-4.5,-4.6,11.5)) ;
#22321=CARTESIAN_POINT('Origin',(4.5,-4.9,11.5)) ;
#22322=CARTESIAN_POINT('',(4.5,-5.2,13.5)) ;
#22323=CARTESIAN_POINT('',(4.5,-5.2,9.5)) ;
#22324=CARTESIAN_POINT('',(4.5,-5.2,11.5)) ;
#22325=CARTESIAN_POINT('',(4.5,-4.9,9.5)) ;
#22326=CARTESIAN_POINT('',(4.5,-4.9,13.5)) ;
#22327=CARTESIAN_POINT('Origin',(0.,-4.9,13.5)) ;
#22328=CARTESIAN_POINT('',(-4.5,-5.2,13.5)) ;
#22329=CARTESIAN_POINT('',(-4.5,-4.9,13.5)) ;
#22330=CARTESIAN_POINT('',(0.,-5.2,13.5)) ;
#22331=CARTESIAN_POINT('Origin',(0.,-4.9,9.5)) ;
#22332=CARTESIAN_POINT('',(-4.5,-5.2,9.5)) ;
#22333=CARTESIAN_POINT('',(0.,-5.2,9.5)) ;
#22334=CARTESIAN_POINT('',(-4.5,-4.9,9.5)) ;
#22335=CARTESIAN_POINT('Origin',(0.,-5.2,11.5)) ;
#22336=CARTESIAN_POINT('',(-4.5,-5.2,11.5)) ;
#22337=CARTESIAN_POINT('Origin',(-4.5,-4.9,11.5)) ;
#24553=UNCERTAINTY_MEASURE_WITH_UNIT(LENGTH_MEASURE(0.001),#24629,
'DISTANCE_ACCURACY_VALUE',
'Maximum model space distance between geometric entities at asserted c
onnectivities') ;
#24580=UNCERTAINTY_MEASURE_WITH_UNIT(LENGTH_MEASURE(0.001),#24629,
'DISTANCE_ACCURACY_VALUE',
'Maximum model space distance between geometric entities at asserted c
onnectivities') ;
#24601=(
GEOMETRIC_REPRESENTATION_CONTEXT(3)
GLOBAL_UNCERTAINTY_ASSIGNED_CONTEXT((#24553))
GLOBAL_UNIT_ASSIGNED_CONTEXT((#24629,#24631,#24632))
REPRESENTATION_CONTEXT('','3D')
) ;
#24628=(
GEOMETRIC_REPRESENTATION_CONTEXT(3)
GLOBAL_UNCERTAINTY_ASSIGNED_CONTEXT((#24580))
GLOBAL_UNIT_ASSIGNED_CONTEXT((#24629,#24631,#24632))
REPRESENTATION_CONTEXT('','3D')
) ;
#24629=(
LENGTH_UNIT()
NAMED_UNIT(*)
SI_UNIT(.CENTI.,.METRE.)
) ;
#24631=(
NAMED_UNIT(*)
PLANE_ANGLE_UNIT()
SI_UNIT($,.RADIAN.)
) ;
#24632=(
NAMED_UNIT(*)
SI_UNIT($,.STERADIAN.)
SOLID_ANGLE_UNIT()
) ;
#24653=SHAPE_DEFINITION_REPRESENTATION(#24700,#24811) ;
#24700=PRODUCT_DEFINITION_SHAPE('',$,#24859) ;
#24811=SHAPE_REPRESENTATION('',(#14802),#24601) ;
#24838=PRODUCT_DEFINITION_CONTEXT('part definition',#24981,'design') ;
#24859=PRODUCT_DEFINITION('MOUNTING_BRACKET_FLANGE',
'MOUNTING_BRACKET_FLANGE',#24906,#24838) ;
#24906=PRODUCT_DEFINITION_FORMATION('',$,#25003) ;
#24981=APPLICATION_CONTEXT(
'Core Data for Automotive Mechanical Design Process') ;
#24982=PRODUCT_CONTEXT('part definition',#24981,'mechanical') ;
#25003=PRODUCT('MOUNTING_BRACKET_FLANGE','MOUNTING_BRACKET_FLANGE',$,(#24982)) ;
#25037=PRESENTATION_STYLE_ASSIGNMENT((#25047)) ;
#25047=SURFACE_STYLE_USAGE(.BOTH.,#25057) ;
#25057=SURFACE_SIDE_STYLE('',(#25067)) ;
#25067=SURFACE_STYLE_FILL_AREA(#25077) ;
#25077=FILL_AREA_STYLE('Steel - Galvanized (Small)',(#25087)) ;
#25087=FILL_AREA_STYLE_COLOUR('Steel - Galvanized (Small)',#25097) ;
#25097=COLOUR_RGB('Steel - Galvanized (Small)', 0.31764706, 0.68627451, 0.89019608) ;
ENDSEC;
END-ISO-10303-21;
